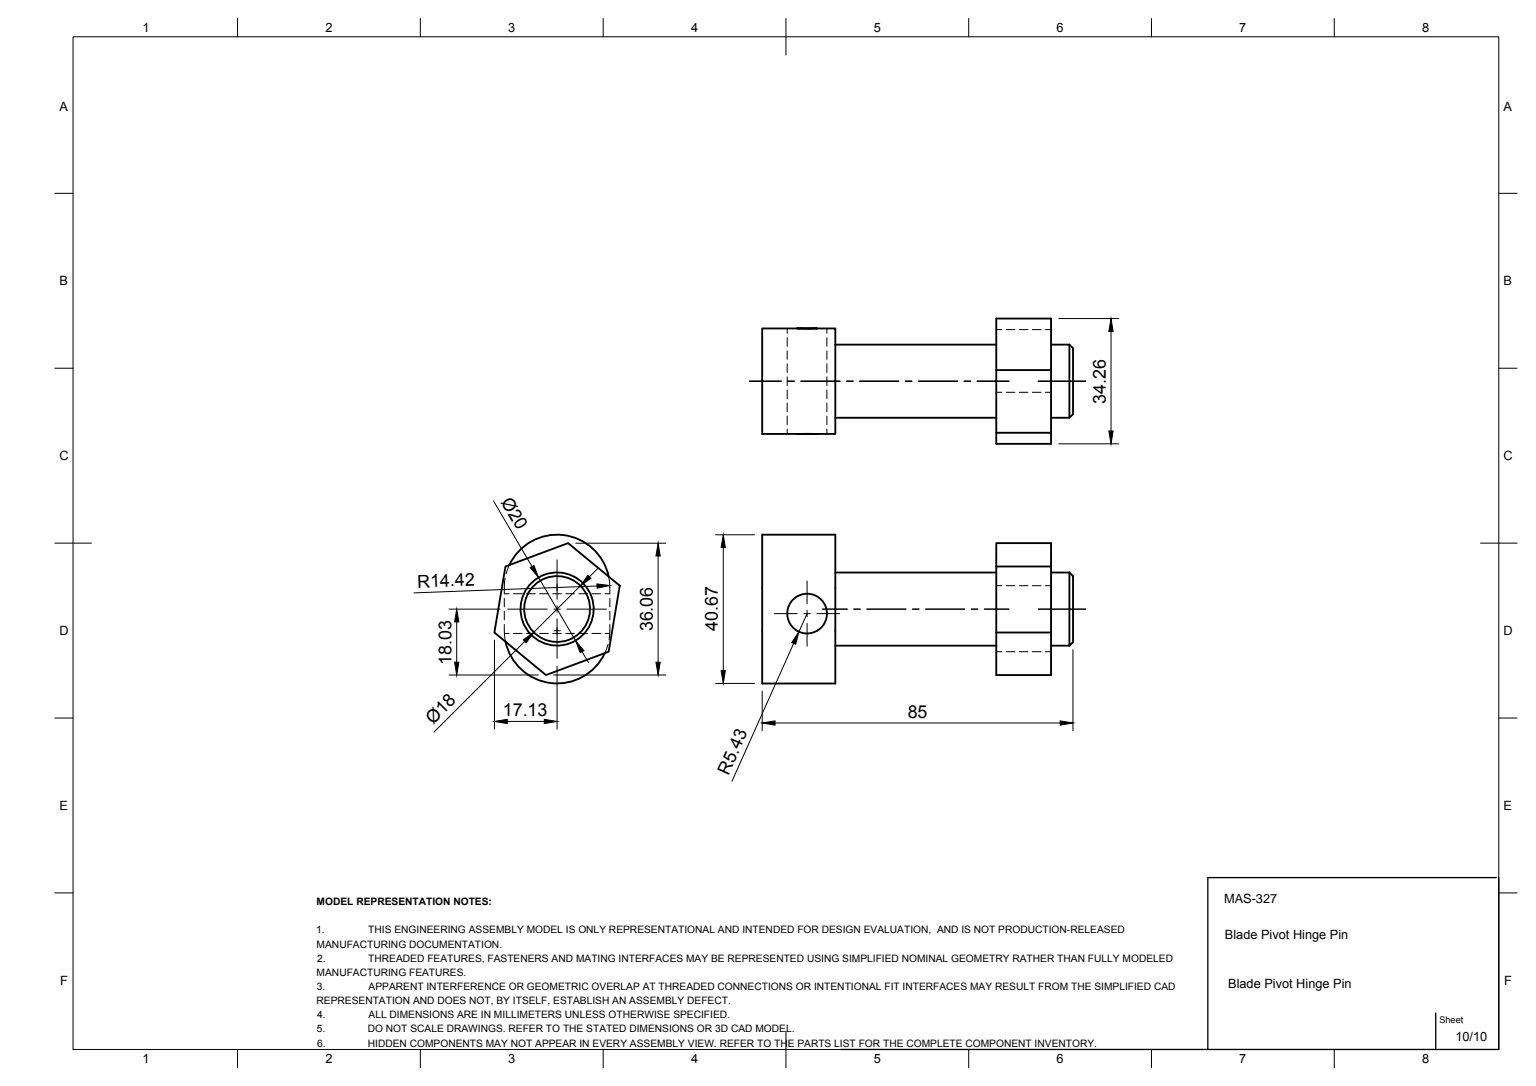
ISO-10303-21;
HEADER;
FILE_DESCRIPTION (('STEP AP214'),
    '1' );
FILE_NAME ('Blade Pivot Hinge Pin.step',
    '2026-10-06T22:16:42',
    ( '' ),
    ( '' ),
    'SwSTEP 2.0',
    'SolidWorks 2025',
    '' );
FILE_SCHEMA (( 'AUTOMOTIVE_DESIGN' ));
ENDSEC;

DATA;
#32=VERTEX_POINT ( 'NONE', #9176 ) ;
#71=CIRCLE ( 'NONE', #14485, 14.42424326798555434 ) ;
#91=AXIS2_PLACEMENT_3D ( 'NONE', #5623, #16792, #1591 ) ;
#93=ORIENTED_EDGE ( 'NONE', *, *, #5608, .T. ) ;
#149=ORIENTED_EDGE ( 'NONE', *, *, #5345, .F. ) ;
#155=FILL_AREA_STYLE_COLOUR ( '', #636 ) ;
#175=VERTEX_POINT ( 'NONE', #1443 ) ;
#180=CARTESIAN_POINT ( 'NONE',  ( 165.8083469658213005, 192.9029763258799335, -44.99999999999997158 ) ) ;
#237=DIRECTION ( 'NONE',  ( 0.000000000000000000, 0.000000000000000000, 1.000000000000000000 ) ) ;
#291=CARTESIAN_POINT ( 'NONE',  ( 163.1026836591718734, 192.4288937294299160, 34.00000000000001421 ) ) ;
#292=CARTESIAN_POINT ( 'NONE',  ( 163.3401611601854029, 191.7221236944928364, 21.73429951086134082 ) ) ;
#367=ORIENTED_EDGE ( 'NONE', *, *, #11936, .F. ) ;
#369=EDGE_LOOP ( 'NONE', ( #21532, #16154, #367, #8720 ) ) ;
#378=LINE ( 'NONE', #18569, #11533 ) ;
#385=CARTESIAN_POINT ( 'NONE',  ( 147.5268905834513475, 193.0332408774651185, -50.99999999999998579 ) ) ;
#410=CARTESIAN_POINT ( 'NONE',  ( 145.5008360144876747, 198.5836349573982886, 14.00000000000001776 ) ) ;
#412=LINE ( 'NONE', #12191, #11898 ) ;
#430=CYLINDRICAL_SURFACE ( 'NONE', #1907, 10.00000000000000888 ) ;
#439=LINE ( 'NONE', #539, #1132 ) ;
#444=DIRECTION ( 'NONE',  ( -0.000000000000000000, -0.000000000000000000, 1.000000000000000000 ) ) ;
#445=ORIENTED_EDGE ( 'NONE', *, *, #15692, .F. ) ;
#457=LINE ( 'NONE', #7188, #7476 ) ;
#497=VERTEX_POINT ( 'NONE', #9152 ) ;
#520=FACE_OUTER_BOUND ( 'NONE', #589, .T. ) ;
#539=CARTESIAN_POINT ( 'NONE',  ( 138.4989748031516967, 208.9305787985672680, -44.99999999999997158 ) ) ;
#583=VECTOR ( 'NONE', #3604, 1000.000000000000114 ) ;
#589=EDGE_LOOP ( 'NONE', ( #10743, #2541, #5246, #20217, #1667 ) ) ;
#612=VECTOR ( 'NONE', #11258, 1000.000000000000227 ) ;
#636=COLOUR_RGB ( '', 0.72549020, 0.75294118, 0.79215686) ;
#692=DIRECTION ( 'NONE',  ( -1.000000000000000000, 0.000000000000000000, 0.000000000000000000 ) ) ;
#696=DIRECTION ( 'NONE',  ( 0.9999746145782334450, -0.007125320983191549967, 0.000000000000000000 ) ) ;
#707=FACE_OUTER_BOUND ( 'NONE', #3120, .T. ) ;
#743=CARTESIAN_POINT ( 'NONE',  ( 157.5268905834513475, 193.0332408774651185, -50.99999999999998579 ) ) ;
#765=CARTESIAN_POINT ( 'NONE',  ( 136.0032066456581390, 182.5367998656340944, 34.00000000000001421 ) ) ;
#804=CYLINDRICAL_SURFACE ( 'NONE', #5889, 10.00000000000000888 ) ;
#883=FACE_OUTER_BOUND ( 'NONE', #16754, .T. ) ;
#884=LINE ( 'NONE', #9271, #9392 ) ;
#886=DIRECTION ( 'NONE',  ( -1.000000000000000000, 0.000000000000000000, 0.000000000000000000 ) ) ;
#956=CIRCLE ( 'NONE', #2372, 5.425037101889737201 ) ;
#973=CARTESIAN_POINT ( 'NONE',  ( 156.5548063637509415, 177.1359029563629406, -29.99999999999997868 ) ) ;
#980=EDGE_CURVE ( 'NONE', #32, #12851, #19907, .T. ) ;
#1057=CARTESIAN_POINT ( 'NONE',  ( 147.5268905834513475, 193.0332408774651185, -50.99999999999998579 ) ) ;
#1061=ADVANCED_FACE ( 'NONE', ( #2071, #9126 ), #20695, .F. ) ;
#1115=ADVANCED_FACE ( 'NONE', ( #520 ), #15825, .T. ) ;
#1122=LINE ( 'NONE', #12914, #6565 ) ;
#1123=VECTOR ( 'NONE', #20357, 1000.000000000000000 ) ;
#1132=VECTOR ( 'NONE', #18955, 1000.000000000000114 ) ;
#1210=FACE_OUTER_BOUND ( 'NONE', #15224, .T. ) ;
#1211=VECTOR ( 'NONE', #3473, 1000.000000000000000 ) ;
#1227=VERTEX_POINT ( 'NONE', #4367 ) ;
#1256=EDGE_CURVE ( 'NONE', #2768, #6341, #16602, .T. ) ;
#1325=ORIENTED_EDGE ( 'NONE', *, *, #18533, .F. ) ;
#1386=EDGE_CURVE ( 'NONE', #6341, #2204, #8241, .T. ) ;
#1395=CYLINDRICAL_SURFACE ( 'NONE', #20750, 14.42424326798555434 ) ;
#1410=PRODUCT_DEFINITION_FORMATION_WITH_SPECIFIED_SOURCE ( 'ANY', '', #14993, .NOT_KNOWN. ) ;
#1418=ORIENTED_EDGE ( 'NONE', *, *, #7944, .F. ) ;
#1420=CARTESIAN_POINT ( 'NONE',  ( 137.5268905834513191, 193.0332408774651185, -29.99999999999997868 ) ) ;
#1429=DIRECTION ( 'NONE',  ( 0.000000000000000000, 0.000000000000000000, -1.000000000000000000 ) ) ;
#1443=CARTESIAN_POINT ( 'NONE',  ( 129.2454342010813662, 193.1635054290503319, -44.99999999999997158 ) ) ;
#1462=EDGE_CURVE ( 'NONE', #9423, #12336, #15502, .T. ) ;
#1473=ORIENTED_EDGE ( 'NONE', *, *, #15351, .T. ) ;
#1537=CARTESIAN_POINT ( 'NONE',  ( 165.8083469658213005, 192.9029763258799335, -44.99999999999997158 ) ) ;
#1561=EDGE_CURVE ( 'NONE', #6540, #20418, #2056, .T. ) ;
#1591=DIRECTION ( 'NONE',  ( -1.000000000000000000, 0.000000000000000000, -0.000000000000000000 ) ) ;
#1613=AXIS2_PLACEMENT_3D ( 'NONE', #14650, #9274, #21390 ) ;
#1667=ORIENTED_EDGE ( 'NONE', *, *, #1675, .T. ) ;
#1675=EDGE_CURVE ( 'NONE', #16415, #5871, #2693, .T. ) ;
#1676=VECTOR ( 'NONE', #18323, 1000.000000000000000 ) ;
#1697=EDGE_CURVE ( 'NONE', #15900, #2204, #8782, .T. ) ;
#1699=VERTEX_POINT ( 'NONE', #2375 ) ;
#1720=SHAPE_REPRESENTATION ( 'Blade Pivot Hinge Pin', ( #12657 ), #4220 ) ;
#1739=ADVANCED_FACE ( 'NONE', ( #20787 ), #16724, .T. ) ;
#1774=ORIENTED_EDGE ( 'NONE', *, *, #5185, .T. ) ;
#1812=CARTESIAN_POINT ( 'NONE',  ( 156.5548063637509415, 177.1359029563629406, -44.99999999999997158 ) ) ;
#1813=CARTESIAN_POINT ( 'NONE',  ( 147.5268905834513475, 193.0332408774651185, -49.99999999999997158 ) ) ;
#1843=( NAMED_UNIT ( * ) PLANE_ANGLE_UNIT ( ) SI_UNIT ( $, .RADIAN. ) );
#1857=EDGE_CURVE ( 'NONE', #16415, #13585, #20018, .T. ) ;
#1864=CARTESIAN_POINT ( 'NONE',  ( 163.1026836591718734, 192.4288937294299160, 34.00000000000001421 ) ) ;
#1907=AXIS2_PLACEMENT_3D ( 'NONE', #20385, #15625, #15526 ) ;
#1933=VERTEX_POINT ( 'NONE', #7782 ) ;
#1948=VECTOR ( 'NONE', #7134, 1000.000000000000227 ) ;
#1991=AXIS2_PLACEMENT_3D ( 'NONE', #5809, #10997, #17814 ) ;
#1993=CIRCLE ( 'NONE', #19956, 14.42424326798555434 ) ;
#2004=LINE ( 'NONE', #20415, #5529 ) ;
#2031=DIRECTION ( 'NONE',  ( 0.3428981916074316239, -0.9393725726208708160, -0.000000000000000000 ) ) ;
#2056=LINE ( 'NONE', #11750, #15327 ) ;
#2071=FACE_OUTER_BOUND ( 'NONE', #10103, .T. ) ;
#2081=CARTESIAN_POINT ( 'NONE',  ( 156.5548063637509415, 177.1359029563629406, -44.99999999999997158 ) ) ;
#2096=DIRECTION ( 'NONE',  ( -0.3428981916074316239, 0.9393725726208708160, 0.000000000000000000 ) ) ;
#2105=ADVANCED_FACE ( 'NONE', ( #21775 ), #12052, .F. ) ;
#2124=ORIENTED_EDGE ( 'NONE', *, *, #21477, .F. ) ;
#2204=VERTEX_POINT ( 'NONE', #13707 ) ;
#2211=EDGE_CURVE ( 'NONE', #13585, #16648, #10200, .T. ) ;
#2284=ADVANCED_FACE ( 'NONE', ( #1210 ), #7217, .T. ) ;
#2303=PLANE ( 'NONE',  #16261 ) ;
#2304=EDGE_CURVE ( 'NONE', #15900, #1933, #11111, .T. ) ;
#2319=DIRECTION ( 'NONE',  ( -1.000000000000000000, 0.000000000000000000, 0.000000000000000000 ) ) ;
#2346=DIRECTION ( 'NONE',  ( -0.007125320983191549967, -0.9999746145782334450, 0.000000000000000000 ) ) ;
#2372=AXIS2_PLACEMENT_3D ( 'NONE', #17761, #9738, #18092 ) ;
#2375=CARTESIAN_POINT ( 'NONE',  ( 136.0032066456581674, 182.5367998656340944, 18.98992973508700643 ) ) ;
#2394=AXIS2_PLACEMENT_3D ( 'NONE', #3060, #9903, #4940 ) ;
#2403=CARTESIAN_POINT ( 'NONE',  ( 0.000000000000000000, 0.000000000000000000, 0.000000000000000000 ) ) ;
#2443=ORIENTED_EDGE ( 'NONE', *, *, #20870, .T. ) ;
#2461=ORIENTED_EDGE ( 'NONE', *, *, #21477, .T. ) ;
#2463=CARTESIAN_POINT ( 'NONE',  ( 138.2733499813809885, 177.2661675079481540, -29.99999999999997868 ) ) ;
#2488=ORIENTED_EDGE ( 'NONE', *, *, #1675, .F. ) ;
#2499=LINE ( 'NONE', #743, #5251 ) ;
#2541=ORIENTED_EDGE ( 'NONE', *, *, #10210, .T. ) ;
#2569=ORIENTED_EDGE ( 'NONE', *, *, #16333, .F. ) ;
#2573=LINE ( 'NONE', #5773, #19594 ) ;
#2583=CARTESIAN_POINT ( 'NONE',  ( 136.1559806577886036, 182.1353248703794350, 23.62031749096655275 ) ) ;
#2667=ORIENTED_EDGE ( 'NONE', *, *, #5537, .T. ) ;
#2674=CARTESIAN_POINT ( 'NONE',  ( 147.5268905834513475, 193.0332408774651185, -44.99999999999997158 ) ) ;
#2693=LINE ( 'NONE', #7565, #6529 ) ;
#2715=AXIS2_PLACEMENT_3D ( 'NONE', #9298, #2346, #696 ) ;
#2768=VERTEX_POINT ( 'NONE', #5833 ) ;
#2806=DIRECTION ( 'NONE',  ( -0.000000000000000000, -0.000000000000000000, -1.000000000000000000 ) ) ;
#2887=PLANE ( 'NONE',  #7204 ) ;
#2914=DIRECTION ( 'NONE',  ( 0.9393725726208708160, 0.3428981916074316794, -0.000000000000000000 ) ) ;
#3026=DIRECTION ( 'NONE',  ( -0.4938165983075539223, 0.8695660798558991766, 0.000000000000000000 ) ) ;
#3060=CARTESIAN_POINT ( 'NONE',  ( 147.5268905834513475, 193.0332408774651185, 14.00000000000001776 ) ) ;
#3120=EDGE_LOOP ( 'NONE', ( #3971, #3699, #6691, #12257 ) ) ;
#3133=CARTESIAN_POINT ( 'NONE',  ( 156.5548063637509415, 177.1359029563629406, -29.99999999999997868 ) ) ;
#3229=EDGE_CURVE ( 'NONE', #12336, #6852, #3737, .T. ) ;
#3237=ORIENTED_EDGE ( 'NONE', *, *, #5860, .T. ) ;
#3248=SURFACE_STYLE_USAGE ( .BOTH. , #6887 ) ;
#3260=EDGE_LOOP ( 'NONE', ( #6641, #16425, #15413, #4890, #20873, #14634, #7629 ) ) ;
#3285=EDGE_CURVE ( 'NONE', #9423, #15135, #21427, .T. ) ;
#3330=EDGE_CURVE ( 'NONE', #12794, #19825, #7275, .T. ) ;
#3384=CARTESIAN_POINT ( 'NONE',  ( 163.1026836591718734, 192.4288937294299160, 34.00000000000001421 ) ) ;
#3404=AXIS2_PLACEMENT_3D ( 'NONE', #14232, #14124, #7424 ) ;
#3406=ORIENTED_EDGE ( 'NONE', *, *, #16132, .F. ) ;
#3407=CARTESIAN_POINT ( 'NONE',  ( 137.5268905834513191, 193.0332408774651185, 14.00000000000001776 ) ) ;
#3420=DIRECTION ( 'NONE',  ( -0.9393725726208708160, -0.3428981916074316239, 0.000000000000000000 ) ) ;
#3464=CIRCLE ( 'NONE', #2394, 10.00000000000000888 ) ;
#3467=EDGE_CURVE ( 'NONE', #5871, #8301, #1993, .T. ) ;
#3473=DIRECTION ( 'NONE',  ( 0.7071067811865456854, 0.000000000000000000, 0.7071067811865493491 ) ) ;
#3497=CARTESIAN_POINT ( 'NONE',  ( 129.2454342010813662, 193.1635054290503319, -29.99999999999997868 ) ) ;
#3540=ORIENTED_EDGE ( 'NONE', *, *, #18228, .F. ) ;
#3553=PRODUCT_DEFINITION_CONTEXT ( 'detailed design', #11668, 'design' ) ;
#3576=FACE_BOUND ( 'NONE', #8312, .T. ) ;
#3587=LINE ( 'NONE', #17017, #10630 ) ;
#3604=DIRECTION ( 'NONE',  ( -0.3428981916074316239, 0.9393725726208708160, 0.000000000000000000 ) ) ;
#3633=PLANE ( 'NONE',  #19511 ) ;
#3646=EDGE_CURVE ( 'NONE', #12851, #32, #3464, .T. ) ;
#3661=CARTESIAN_POINT ( 'NONE',  ( 138.5268905834513191, 193.0332408774651185, -50.99999999999998579 ) ) ;
#3699=ORIENTED_EDGE ( 'NONE', *, *, #14722, .F. ) ;
#3701=ORIENTED_EDGE ( 'NONE', *, *, #15830, .F. ) ;
#3737=LINE ( 'NONE', #2081, #14645 ) ;
#3785=AXIS2_PLACEMENT_3D ( 'NONE', #1057, #19682, #21452 ) ;
#3810=AXIS2_PLACEMENT_3D ( 'NONE', #10387, #6975, #17304 ) ;
#3856=AXIS2_PLACEMENT_3D ( 'NONE', #9588, #21159, #4387 ) ;
#3861=ORIENTED_EDGE ( 'NONE', *, *, #15351, .F. ) ;
#3895=FACE_OUTER_BOUND ( 'NONE', #4743, .T. ) ;
#3906=ORIENTED_EDGE ( 'NONE', *, *, #980, .F. ) ;
#3921=CARTESIAN_POINT ( 'NONE',  ( 163.3215298332769407, 191.7840731147956319, 22.69574685642843193 ) ) ;
#3935=EDGE_CURVE ( 'NONE', #14777, #14246, #412, .T. ) ;
#3971=ORIENTED_EDGE ( 'NONE', *, *, #5276, .T. ) ;
#4000=CARTESIAN_POINT ( 'NONE',  ( 131.9510975077307933, 193.6375880255003779, 14.00000000000001776 ) ) ;
#4008=LINE ( 'NONE', #4219, #19072 ) ;
#4049=EDGE_LOOP ( 'NONE', ( #10376, #18796, #8509, #20618 ) ) ;
#4074=ORIENTED_EDGE ( 'NONE', *, *, #5608, .F. ) ;
#4094=ORIENTED_EDGE ( 'NONE', *, *, #8231, .T. ) ;
#4136=CIRCLE ( 'NONE', #4292, 10.00000000000000888 ) ;
#4158=ORIENTED_EDGE ( 'NONE', *, *, #17674, .F. ) ;
#4219=CARTESIAN_POINT ( 'NONE',  ( 136.0032066456581390, 182.5367998656340944, 34.00000000000001421 ) ) ;
#4220=( GEOMETRIC_REPRESENTATION_CONTEXT ( 3 ) GLOBAL_UNCERTAINTY_ASSIGNED_CONTEXT ( ( #20336 ) ) GLOBAL_UNIT_ASSIGNED_CONTEXT ( ( #21579, #1843, #6470 ) ) REPRESENTATION_CONTEXT ( 'NONE', 'WORKASPACE' ) );
#4251=ORIENTED_EDGE ( 'NONE', *, *, #3330, .F. ) ;
#4255=DIRECTION ( 'NONE',  ( -1.000000000000000000, 0.000000000000000000, -0.000000000000000000 ) ) ;
#4261=DIRECTION ( 'NONE',  ( -1.000000000000000000, 0.000000000000000000, 0.000000000000000000 ) ) ;
#4292=AXIS2_PLACEMENT_3D ( 'NONE', #10711, #17414, #2319 ) ;
#4304=ORIENTED_EDGE ( 'NONE', *, *, #7932, .F. ) ;
#4323=VERTEX_POINT ( 'NONE', #4574 ) ;
#4329=DIRECTION ( 'NONE',  ( -1.000000000000000000, 0.000000000000000000, 0.000000000000000000 ) ) ;
#4330=CARTESIAN_POINT ( 'NONE',  ( 165.8083469658213005, 192.9029763258799335, -29.99999999999997868 ) ) ;
#4367=CARTESIAN_POINT ( 'NONE',  ( 138.4989748031516967, 208.9305787985672680, -29.99999999999997868 ) ) ;
#4387=DIRECTION ( 'NONE',  ( -1.000000000000000000, 0.000000000000000000, 0.000000000000000000 ) ) ;
#4463=EDGE_CURVE ( 'NONE', #10265, #14309, #19983, .T. ) ;
#4530=DIRECTION ( 'NONE',  ( 0.4938165983075534227, -0.8695660798558993987, 0.000000000000000000 ) ) ;
#4574=CARTESIAN_POINT ( 'NONE',  ( 159.6377923430271153, 201.9209935688625421, 21.73429951086134082 ) ) ;
#4582=LINE ( 'NONE', #6463, #12990 ) ;
#4597=CARTESIAN_POINT ( 'NONE',  ( 145.5008360144876747, 198.5836349573982886, 34.00000000000001421 ) ) ;
#4627=ORIENTED_EDGE ( 'NONE', *, *, #11087, .T. ) ;
#4658=EDGE_LOOP ( 'NONE', ( #12688, #8306, #8008, #21182 ) ) ;
#4673=CARTESIAN_POINT ( 'NONE',  ( 138.2733499813809885, 177.2661675079481540, -44.99999999999997158 ) ) ;
#4699=CARTESIAN_POINT ( 'NONE',  ( 163.3023584364855196, 191.8436256089667324, 20.54250398750395590 ) ) ;
#4721=DIRECTION ( 'NONE',  ( -0.000000000000000000, -0.000000000000000000, 1.000000000000000000 ) ) ;
#4743=EDGE_LOOP ( 'NONE', ( #19322, #8584, #17876, #20034 ) ) ;
#4817=AXIS2_PLACEMENT_3D ( 'NONE', #11281, #2914, #6327 ) ;
#4829=EDGE_LOOP ( 'NONE', ( #2443, #18990, #4158, #18962 ) ) ;
#4835=CARTESIAN_POINT ( 'NONE',  ( 163.3401611601854029, 191.7221236944928364, 21.73429951086134082 ) ) ;
#4837=ADVANCED_FACE ( 'NONE', ( #707 ), #7440, .F. ) ;
#4860=VERTEX_POINT ( 'NONE', #20125 ) ;
#4890=ORIENTED_EDGE ( 'NONE', *, *, #16132, .T. ) ;
#4930=CARTESIAN_POINT ( 'NONE',  ( 177.7722984847500527, 196.9902717476302882, 21.73429951086134082 ) ) ;
#4940=DIRECTION ( 'NONE',  ( -1.000000000000000000, 0.000000000000000000, 0.000000000000000000 ) ) ;
#4979=PRODUCT_DEFINITION_SHAPE ( 'NONE', 'NONE',  #8803 ) ;
#4988=DIRECTION ( 'NONE',  ( -0.000000000000000000, -0.000000000000000000, 1.000000000000000000 ) ) ;
#5012=VECTOR ( 'NONE', #444, 1000.000000000000000 ) ;
#5015=CARTESIAN_POINT ( 'NONE',  ( 163.1026836591718734, 192.4288937294299160, 24.47866928663567521 ) ) ;
#5020=CARTESIAN_POINT ( 'NONE',  ( 165.8083469658213005, 192.9029763258799335, -29.99999999999997868 ) ) ;
#5033=ADVANCED_FACE ( 'NONE', ( #10629 ), #804, .T. ) ;
#5052=CARTESIAN_POINT ( 'NONE',  ( 147.5268905834513475, 193.0332408774651185, 14.00000000000001776 ) ) ;
#5095=LINE ( 'NONE', #8408, #6858 ) ;
#5099=ADVANCED_FACE ( 'NONE', ( #20980 ), #15578, .F. ) ;
#5118=( LENGTH_UNIT ( ) NAMED_UNIT ( * ) SI_UNIT ( .MILLI., .METRE. ) );
#5151=DIRECTION ( 'NONE',  ( 0.000000000000000000, 0.000000000000000000, 1.000000000000000000 ) ) ;
#5185=EDGE_CURVE ( 'NONE', #1933, #1699, #956, .T. ) ;
#5221=EDGE_LOOP ( 'NONE', ( #5749, #9154, #20697, #12554 ) ) ;
#5242=CARTESIAN_POINT ( 'NONE',  ( 131.9510975077307933, 193.6375880255003779, 34.00000000000001421 ) ) ;
#5246=ORIENTED_EDGE ( 'NONE', *, *, #5344, .T. ) ;
#5251=VECTOR ( 'NONE', #20916, 1000.000000000000000 ) ;
#5276=EDGE_CURVE ( 'NONE', #10216, #1227, #21197, .T. ) ;
#5324=ORIENTED_EDGE ( 'NONE', *, *, #1386, .T. ) ;
#5344=EDGE_CURVE ( 'NONE', #5609, #497, #9420, .T. ) ;
#5345=EDGE_CURVE ( 'NONE', #1699, #16648, #2004, .T. ) ;
#5374=EDGE_LOOP ( 'NONE', ( #20914, #1325, #7393, #12040 ) ) ;
#5417=AXIS2_PLACEMENT_3D ( 'NONE', #4597, #10012, #13315 ) ;
#5437=EDGE_CURVE ( 'NONE', #175, #10216, #6533, .T. ) ;
#5468=VERTEX_POINT ( 'NONE', #13363 ) ;
#5475=VECTOR ( 'NONE', #2031, 1000.000000000000114 ) ;
#5529=VECTOR ( 'NONE', #18760, 1000.000000000000000 ) ;
#5537=EDGE_CURVE ( 'NONE', #11247, #32, #19298, .T. ) ;
#5563=CARTESIAN_POINT ( 'NONE',  ( 163.3401611601853745, 191.7221236944928364, 22.21121901686272793 ) ) ;
#5608=EDGE_CURVE ( 'NONE', #19825, #12794, #4136, .T. ) ;
#5609=VERTEX_POINT ( 'NONE', #14108 ) ;
#5610=CARTESIAN_POINT ( 'NONE',  ( 138.4989748031516967, 208.9305787985672680, -44.99999999999997158 ) ) ;
#5623=CARTESIAN_POINT ( 'NONE',  ( 0.000000000000000000, 0.000000000000000000, -44.99999999999997158 ) ) ;
#5631=ADVANCED_FACE ( 'NONE', ( #8948 ), #15655, .F. ) ;
#5651=CARTESIAN_POINT ( 'NONE',  ( 136.0451547902032701, 182.4218825594992950, 19.19853326693791473 ) ) ;
#5669=EDGE_CURVE ( 'NONE', #8397, #19825, #457, .T. ) ;
#5740=EDGE_LOOP ( 'NONE', ( #11373, #10373 ) ) ;
#5749=ORIENTED_EDGE ( 'NONE', *, *, #15830, .T. ) ;
#5755=CARTESIAN_POINT ( 'NONE',  ( 136.1510593568410172, 182.1483534088744420, 19.85643285628697541 ) ) ;
#5773=CARTESIAN_POINT ( 'NONE',  ( 174.0518276614676267, 207.1825338655619646, 21.73429951086134082 ) ) ;
#5792=ORIENTED_EDGE ( 'NONE', *, *, #1857, .F. ) ;
#5809=CARTESIAN_POINT ( 'NONE',  ( 156.7804311855217065, 208.8003142469820830, -44.99999999999997158 ) ) ;
#5833=CARTESIAN_POINT ( 'NONE',  ( 163.1026836591718734, 192.4288937294299160, 18.98992973508700643 ) ) ;
#5844=ORIENTED_EDGE ( 'NONE', *, *, #1697, .T. ) ;
#5860=EDGE_CURVE ( 'NONE', #4860, #13585, #71, .T. ) ;
#5871=VERTEX_POINT ( 'NONE', #8794 ) ;
#5889=AXIS2_PLACEMENT_3D ( 'NONE', #15788, #19320, #17334 ) ;
#5943=DIRECTION ( 'NONE',  ( -1.000000000000000000, 0.000000000000000000, 0.000000000000000000 ) ) ;
#6000=PRODUCT_CONTEXT ( 'NONE', #15354, 'mechanical' ) ;
#6053=DIRECTION ( 'NONE',  ( 0.000000000000000000, 0.000000000000000000, -1.000000000000000000 ) ) ;
#6056=DIRECTION ( 'NONE',  ( 0.000000000000000000, 0.000000000000000000, 1.000000000000000000 ) ) ;
#6083=CARTESIAN_POINT ( 'NONE',  ( 129.2454342010813662, 193.1635054290503319, -29.99999999999997868 ) ) ;
#6130=AXIS2_PLACEMENT_3D ( 'NONE', #14301, #17819, #17606 ) ;
#6202=VECTOR ( 'NONE', #20458, 1000.000000000000227 ) ;
#6261=ORIENTED_EDGE ( 'NONE', *, *, #1857, .T. ) ;
#6327=DIRECTION ( 'NONE',  ( 0.3428981916074309577, -0.9393725726208709270, 0.000000000000000000 ) ) ;
#6341=VERTEX_POINT ( 'NONE', #292 ) ;
#6368=DIRECTION ( 'NONE',  ( 0.000000000000000000, 0.000000000000000000, 1.000000000000000000 ) ) ;
#6379=LINE ( 'NONE', #13108, #20764 ) ;
#6417=CYLINDRICAL_SURFACE ( 'NONE', #6993, 10.00000000000000888 ) ;
#6437=EDGE_CURVE ( 'NONE', #8301, #18099, #15396, .T. ) ;
#6463=CARTESIAN_POINT ( 'NONE',  ( 138.4989748031516967, 208.9305787985672680, -29.99999999999997868 ) ) ;
#6470=( NAMED_UNIT ( * ) SI_UNIT ( $, .STERADIAN. ) SOLID_ANGLE_UNIT ( ) );
#6484=AXIS2_PLACEMENT_3D ( 'NONE', #21065, #6056, #12893 ) ;
#6499=FACE_OUTER_BOUND ( 'NONE', #5374, .T. ) ;
#6529=VECTOR ( 'NONE', #12728, 1000.000000000000114 ) ;
#6533=LINE ( 'NONE', #13253, #1676 ) ;
#6540=VERTEX_POINT ( 'NONE', #12509 ) ;
#6554=SURFACE_STYLE_FILL_AREA ( #18456 ) ;
#6565=VECTOR ( 'NONE', #4530, 1000.000000000000114 ) ;
#6608=CARTESIAN_POINT ( 'NONE',  ( 159.0505745212445561, 203.5296818892961994, 14.00000000000001776 ) ) ;
#6641=ORIENTED_EDGE ( 'NONE', *, *, #6437, .T. ) ;
#6657=CARTESIAN_POINT ( 'NONE',  ( 156.7804311855217065, 208.8003142469820830, -29.99999999999997868 ) ) ;
#6671=ORIENTED_EDGE ( 'NONE', *, *, #9508, .T. ) ;
#6681=CARTESIAN_POINT ( 'NONE',  ( 136.0032066456581390, 182.5367998656340944, 14.00000000000001776 ) ) ;
#6690=CARTESIAN_POINT ( 'NONE',  ( 161.4980277546683283, 196.8248625098966897, 21.73429951086134082 ) ) ;
#6691=ORIENTED_EDGE ( 'NONE', *, *, #14114, .F. ) ;
#6707=CARTESIAN_POINT ( 'NONE',  ( 163.3167426812955227, 191.7976672453297624, 20.78115173001200944 ) ) ;
#6723=ORIENTED_EDGE ( 'NONE', *, *, #5537, .F. ) ;
#6752=ORIENTED_EDGE ( 'NONE', *, *, #5669, .T. ) ;
#6763=CARTESIAN_POINT ( 'NONE',  ( 145.5008360144876747, 198.5836349573982886, 34.00000000000001421 ) ) ;
#6787=DIRECTION ( 'NONE',  ( -0.9999746145782334450, 0.007125320983193088667, 0.000000000000000000 ) ) ;
#6789=EDGE_CURVE ( 'NONE', #20418, #4860, #12398, .T. ) ;
#6851=ORIENTED_EDGE ( 'NONE', *, *, #20870, .F. ) ;
#6852=VERTEX_POINT ( 'NONE', #4673 ) ;
#6858=VECTOR ( 'NONE', #18432, 1000.000000000000000 ) ;
#6871=ADVANCED_FACE ( 'NONE', ( #16456, #3576 ), #15032, .T. ) ;
#6887=SURFACE_SIDE_STYLE ('',( #6554 ) ) ;
#6901=AXIS2_PLACEMENT_3D ( 'NONE', #5052, #8480, #15188 ) ;
#6963=ADVANCED_FACE ( 'NONE', ( #16899 ), #8648, .F. ) ;
#6975=DIRECTION ( 'NONE',  ( -0.000000000000000000, -0.000000000000000000, -1.000000000000000000 ) ) ;
#6993=AXIS2_PLACEMENT_3D ( 'NONE', #21639, #4988, #19869 ) ;
#7002=DIRECTION ( 'NONE',  ( 0.3428981916074309577, -0.9393725726208709270, 0.000000000000000000 ) ) ;
#7050=DIRECTION ( 'NONE',  ( 0.000000000000000000, 0.000000000000000000, 1.000000000000000000 ) ) ;
#7102=MANIFOLD_SOLID_BREP ( 'Chamfer1', #13383 ) ;
#7125=VECTOR ( 'NONE', #11815, 1000.000000000000000 ) ;
#7126=CIRCLE ( 'NONE', #15222, 10.00000000000000888 ) ;
#7134=DIRECTION ( 'NONE',  ( -0.5061580162706792452, -0.8624407588727069918, 0.000000000000000000 ) ) ;
#7188=CARTESIAN_POINT ( 'NONE',  ( 137.5268905834513191, 193.0332408774651185, -50.99999999999998579 ) ) ;
#7204=AXIS2_PLACEMENT_3D ( 'NONE', #15996, #11152, #16432 ) ;
#7217=CYLINDRICAL_SURFACE ( 'NONE', #20627, 14.42424326798555434 ) ;
#7224=DIRECTION ( 'NONE',  ( -0.000000000000000000, -0.000000000000000000, -1.000000000000000000 ) ) ;
#7228=ADVANCED_FACE ( 'NONE', ( #6499 ), #12566, .F. ) ;
#7242=CARTESIAN_POINT ( 'NONE',  ( 136.2768881589198600, 181.8432453435729883, 21.97307119874763259 ) ) ;
#7275=CIRCLE ( 'NONE', #19574, 10.00000000000000888 ) ;
#7329=DIRECTION ( 'NONE',  ( -0.000000000000000000, -0.000000000000000000, -1.000000000000000000 ) ) ;
#7348=EDGE_CURVE ( 'NONE', #14309, #10265, #16864, .T. ) ;
#7393=ORIENTED_EDGE ( 'NONE', *, *, #1462, .F. ) ;
#7424=DIRECTION ( 'NONE',  ( 1.000000000000000000, 0.000000000000000000, 0.000000000000000000 ) ) ;
#7433=ORIENTED_EDGE ( 'NONE', *, *, #7932, .T. ) ;
#7440=PLANE ( 'NONE',  #12589 ) ;
#7452=CARTESIAN_POINT ( 'NONE',  ( 163.2639715594360155, 191.9628544139417841, 23.38668371770654275 ) ) ;
#7476=VECTOR ( 'NONE', #17735, 1000.000000000000000 ) ;
#7500=ADVANCED_FACE ( 'NONE', ( #8705 ), #3633, .F. ) ;
#7539=UNCERTAINTY_MEASURE_WITH_UNIT (LENGTH_MEASURE( 1.000000000000000082E-05 ), #5118, 'distance_accuracy_value', 'NONE');
#7543=EDGE_LOOP ( 'NONE', ( #4627, #9285 ) ) ;
#7554=CARTESIAN_POINT ( 'NONE',  ( 156.7804311855217065, 208.8003142469820830, -29.99999999999997868 ) ) ;
#7565=CARTESIAN_POINT ( 'NONE',  ( 136.0032066456581390, 182.5367998656340944, 34.00000000000001421 ) ) ;
#7585=AXIS2_PLACEMENT_3D ( 'NONE', #12636, #19357, #4255 ) ;
#7623=DIRECTION ( 'NONE',  ( -0.000000000000000000, -0.000000000000000000, -1.000000000000000000 ) ) ;
#7629=ORIENTED_EDGE ( 'NONE', *, *, #10210, .F. ) ;
#7645=ADVANCED_FACE ( 'NONE', ( #21259 ), #15952, .F. ) ;
#7767=ORIENTED_EDGE ( 'NONE', *, *, #20655, .F. ) ;
#7769=DIRECTION ( 'NONE',  ( -0.000000000000000000, -0.000000000000000000, 1.000000000000000000 ) ) ;
#7770=DIRECTION ( 'NONE',  ( -0.5061580162706792452, -0.8624407588727069918, 0.000000000000000000 ) ) ;
#7782=CARTESIAN_POINT ( 'NONE',  ( 132.5383153295133809, 192.0288997050666921, 21.73429951086134082 ) ) ;
#7906=DIRECTION ( 'NONE',  ( 0.9999746145782334450, -0.007125320983191549967, 0.000000000000000000 ) ) ;
#7932=EDGE_CURVE ( 'NONE', #16648, #6540, #18152, .T. ) ;
#7944=EDGE_CURVE ( 'NONE', #497, #16415, #20983, .T. ) ;
#7947=VECTOR ( 'NONE', #15174, 1000.000000000000341 ) ;
#8008=ORIENTED_EDGE ( 'NONE', *, *, #3229, .F. ) ;
#8068=ORIENTED_EDGE ( 'NONE', *, *, #6789, .F. ) ;
#8231=EDGE_CURVE ( 'NONE', #2768, #4323, #11182, .T. ) ;
#8241=LINE ( 'NONE', #4930, #7947 ) ;
#8249=DIRECTION ( 'NONE',  ( 0.000000000000000000, 0.000000000000000000, 1.000000000000000000 ) ) ;
#8301=VERTEX_POINT ( 'NONE', #9552 ) ;
#8306=ORIENTED_EDGE ( 'NONE', *, *, #12097, .F. ) ;
#8312=EDGE_LOOP ( 'NONE', ( #4251, #4074 ) ) ;
#8333=DIRECTION ( 'NONE',  ( 0.9393725726208708160, 0.3428981916074316794, -0.000000000000000000 ) ) ;
#8367=CARTESIAN_POINT ( 'NONE',  ( 157.5268905834513475, 193.0332408774651185, -44.99999999999997158 ) ) ;
#8397=VERTEX_POINT ( 'NONE', #21674 ) ;
#8400=ORIENTED_EDGE ( 'NONE', *, *, #2211, .T. ) ;
#8408=CARTESIAN_POINT ( 'NONE',  ( 156.5548063637509415, 177.1359029563629406, -44.99999999999997158 ) ) ;
#8440=DIRECTION ( 'NONE',  ( 0.5061580162706794672, 0.8624407588727069918, 0.000000000000000000 ) ) ;
#8442=AXIS2_PLACEMENT_3D ( 'NONE', #1537, #14862, #11666 ) ;
#8480=DIRECTION ( 'NONE',  ( 0.000000000000000000, 0.000000000000000000, -1.000000000000000000 ) ) ;
#8507=ORIENTED_EDGE ( 'NONE', *, *, #2211, .F. ) ;
#8509=ORIENTED_EDGE ( 'NONE', *, *, #20655, .T. ) ;
#8524=LINE ( 'NONE', #6657, #17999 ) ;
#8584=ORIENTED_EDGE ( 'NONE', *, *, #15692, .T. ) ;
#8624=FACE_OUTER_BOUND ( 'NONE', #8885, .T. ) ;
#8648=PLANE ( 'NONE',  #15227 ) ;
#8660=DIRECTION ( 'NONE',  ( 1.000000000000000000, 0.000000000000000000, 0.000000000000000000 ) ) ;
#8670=AXIS2_PLACEMENT_3D ( 'NONE', #9901, #8249, #21697 ) ;
#8705=FACE_OUTER_BOUND ( 'NONE', #3260, .T. ) ;
#8720=ORIENTED_EDGE ( 'NONE', *, *, #12097, .T. ) ;
#8782=B_SPLINE_CURVE_WITH_KNOTS ( 'NONE', 3,
 ( #12513, #19452, #2583, #12402, #17785, #17464, #7242, #19134 ),
 .UNSPECIFIED., .F., .F.,
 ( 4, 2, 2, 4 ),
 ( 3.469446951953614189E-18, 0.001432241572422971983, 0.002148362358634445940, 0.002864483144845920114 ),
 .UNSPECIFIED. ) ;
#8794=CARTESIAN_POINT ( 'NONE',  ( 136.0032066456581390, 182.5367998656340944, 34.00000000000001421 ) ) ;
#8803=PRODUCT_DEFINITION ( 'UNKNOWN', '', #1410, #3553 ) ;
#8812=DIRECTION ( 'NONE',  ( -0.9999746145782334450, 0.007125320983193089534, 0.000000000000000000 ) ) ;
#8885=EDGE_LOOP ( 'NONE', ( #1473, #5844, #18307, #9332, #7433, #3406, #10717, #10721, #19853, #16558 ) ) ;
#8936=ADVANCED_FACE ( 'NONE', ( #18090 ), #6417, .T. ) ;
#8948=FACE_OUTER_BOUND ( 'NONE', #19887, .T. ) ;
#8972=CARTESIAN_POINT ( 'NONE',  ( 136.2768881589198884, 181.8432453435730167, 21.73429951086134082 ) ) ;
#8977=ORIENTED_EDGE ( 'NONE', *, *, #16333, .T. ) ;
#9016=ORIENTED_EDGE ( 'NONE', *, *, #11936, .T. ) ;
#9080=DIRECTION ( 'NONE',  ( 0.000000000000000000, 0.000000000000000000, 1.000000000000000000 ) ) ;
#9102=DIRECTION ( 'NONE',  ( -0.9393725726208707050, -0.3428981916074316239, -0.000000000000000000 ) ) ;
#9126=FACE_BOUND ( 'NONE', #7543, .T. ) ;
#9152=CARTESIAN_POINT ( 'NONE',  ( 131.0765927465021434, 198.5836349573982886, 34.00000000000001421 ) ) ;
#9154=ORIENTED_EDGE ( 'NONE', *, *, #3285, .F. ) ;
#9167=FACE_BOUND ( 'NONE', #15105, .T. ) ;
#9170=DIRECTION ( 'NONE',  ( -0.000000000000000000, -0.000000000000000000, 1.000000000000000000 ) ) ;
#9173=ORIENTED_EDGE ( 'NONE', *, *, #1561, .F. ) ;
#9175=ADVANCED_FACE ( 'NONE', ( #8624 ), #19084, .T. ) ;
#9176=CARTESIAN_POINT ( 'NONE',  ( 157.5268905834513475, 193.0332408774651185, 14.00000000000001776 ) ) ;
#9270=( NAMED_UNIT ( * ) PLANE_ANGLE_UNIT ( ) SI_UNIT ( $, .RADIAN. ) );
#9271=CARTESIAN_POINT ( 'NONE',  ( 159.0505745212445561, 203.5296818892961994, 34.00000000000001421 ) ) ;
#9274=DIRECTION ( 'NONE',  ( -0.9393725726208707050, -0.3428981916074317349, 0.000000000000000000 ) ) ;
#9285=ORIENTED_EDGE ( 'NONE', *, *, #20323, .T. ) ;
#9298=CARTESIAN_POINT ( 'NONE',  ( 138.4989748031516967, 208.9305787985672680, -44.99999999999997158 ) ) ;
#9332=ORIENTED_EDGE ( 'NONE', *, *, #5345, .T. ) ;
#9381=DIRECTION ( 'NONE',  ( -0.000000000000000000, -0.000000000000000000, -1.000000000000000000 ) ) ;
#9392=VECTOR ( 'NONE', #7623, 1000.000000000000000 ) ;
#9407=VECTOR ( 'NONE', #9865, 1000.000000000000114 ) ;
#9420=CIRCLE ( 'NONE', #21741, 14.42424326798555434 ) ;
#9423=VERTEX_POINT ( 'NONE', #12894 ) ;
#9474=DIRECTION ( 'NONE',  ( -1.000000000000000000, 0.000000000000000000, 0.000000000000000000 ) ) ;
#9508=EDGE_CURVE ( 'NONE', #5609, #20418, #884, .T. ) ;
#9552=CARTESIAN_POINT ( 'NONE',  ( 163.1026836591718734, 192.4288937294299160, 34.00000000000001421 ) ) ;
#9568=CARTESIAN_POINT ( 'NONE',  ( 163.1026836591718734, 192.4288937294299160, 18.98992973508700643 ) ) ;
#9588=CARTESIAN_POINT ( 'NONE',  ( 147.5268905834513475, 193.0332408774651185, -29.99999999999997868 ) ) ;
#9738=DIRECTION ( 'NONE',  ( -0.9393725726208707050, -0.3428981916074317349, 0.000000000000000000 ) ) ;
#9759=CARTESIAN_POINT ( 'NONE',  ( 145.5008360144876747, 198.5836349573982886, 14.00000000000001776 ) ) ;
#9865=DIRECTION ( 'NONE',  ( -0.9999746145782334450, 0.007125320983193089534, 0.000000000000000000 ) ) ;
#9877=ORIENTED_EDGE ( 'NONE', *, *, #21484, .F. ) ;
#9894=CARTESIAN_POINT ( 'NONE',  ( 163.1866912085270371, 192.1987543186987466, 19.40769008390923389 ) ) ;
#9901=CARTESIAN_POINT ( 'NONE',  ( 149.5529451524149920, 187.4828467975320336, 14.00000000000001776 ) ) ;
#9903=DIRECTION ( 'NONE',  ( 0.000000000000000000, 0.000000000000000000, -1.000000000000000000 ) ) ;
#9922=DIRECTION ( 'NONE',  ( -1.000000000000000000, 0.000000000000000000, 0.000000000000000000 ) ) ;
#9989=DIRECTION ( 'NONE',  ( 0.3428981916074309577, -0.9393725726208709270, 0.000000000000000000 ) ) ;
#9996=ORIENTED_EDGE ( 'NONE', *, *, #20323, .F. ) ;
#9999=ADVANCED_FACE ( 'NONE', ( #20928 ), #11101, .F. ) ;
#10012=DIRECTION ( 'NONE',  ( 0.000000000000000000, 0.000000000000000000, 1.000000000000000000 ) ) ;
#10059=AXIS2_PLACEMENT_3D ( 'NONE', #10870, #17572, #13944 ) ;
#10103=EDGE_LOOP ( 'NONE', ( #16553, #20528, #18905, #19844, #3701, #6851 ) ) ;
#10142=DIRECTION ( 'NONE',  ( 0.3428981916074316239, -0.9393725726208708160, 0.000000000000000000 ) ) ;
#10200=LINE ( 'NONE', #6681, #5475 ) ;
#10210=EDGE_CURVE ( 'NONE', #8301, #5609, #21795, .T. ) ;
#10216=VERTEX_POINT ( 'NONE', #3497 ) ;
#10265=VERTEX_POINT ( 'NONE', #10652 ) ;
#10281=CARTESIAN_POINT ( 'NONE',  ( 136.0032066456581390, 182.5367998656340944, 24.47866928663567521 ) ) ;
#10308=DIRECTION ( 'NONE',  ( 0.8624407588727069918, -0.5061580162706794672, 0.000000000000000000 ) ) ;
#10339=DIRECTION ( 'NONE',  ( -0.000000000000000000, -0.000000000000000000, 1.000000000000000000 ) ) ;
#10344=ORIENTED_EDGE ( 'NONE', *, *, #5185, .F. ) ;
#10368=CIRCLE ( 'NONE', #16339, 10.00000000000000888 ) ;
#10373=ORIENTED_EDGE ( 'NONE', *, *, #7348, .T. ) ;
#10376=ORIENTED_EDGE ( 'NONE', *, *, #5669, .F. ) ;
#10387=CARTESIAN_POINT ( 'NONE',  ( 149.5529451524149920, 187.4828467975320336, 34.00000000000001421 ) ) ;
#10515=MECHANICAL_DESIGN_GEOMETRIC_PRESENTATION_REPRESENTATION('',(#21413),#20361);
#10518=EDGE_CURVE ( 'NONE', #17794, #16883, #18001, .T. ) ;
#10521=CARTESIAN_POINT ( 'NONE',  ( 136.0032066456581674, 182.5367998656340944, 18.98992973508700643 ) ) ;
#10629=FACE_OUTER_BOUND ( 'NONE', #4049, .T. ) ;
#10630=VECTOR ( 'NONE', #15687, 1000.000000000000000 ) ;
#10643=ORIENTED_EDGE ( 'NONE', *, *, #1697, .F. ) ;
#10652=CARTESIAN_POINT ( 'NONE',  ( 156.5268905834513475, 193.0332408774651185, -50.99999999999998579 ) ) ;
#10711=CARTESIAN_POINT ( 'NONE',  ( 147.5268905834513475, 193.0332408774651185, -44.99999999999997158 ) ) ;
#10717=ORIENTED_EDGE ( 'NONE', *, *, #1256, .T. ) ;
#10721=ORIENTED_EDGE ( 'NONE', *, *, #21484, .T. ) ;
#10743=ORIENTED_EDGE ( 'NONE', *, *, #3467, .T. ) ;
#10755=CARTESIAN_POINT ( 'NONE',  ( 163.1026836591718734, 192.4288937294299160, 24.47866928663567521 ) ) ;
#10773=EDGE_CURVE ( 'NONE', #4323, #18099, #19251, .T. ) ;
#10870=CARTESIAN_POINT ( 'NONE',  ( 147.5268905834513475, 193.0332408774651185, -50.99999999999998579 ) ) ;
#10872=SHAPE_DEFINITION_REPRESENTATION ( #4979, #1720 ) ;
#10997=DIRECTION ( 'NONE',  ( -0.8695660798558993987, -0.4938165983075534782, 0.000000000000000000 ) ) ;
#11087=EDGE_CURVE ( 'NONE', #11247, #20292, #18190, .T. ) ;
#11101=PLANE ( 'NONE',  #1991 ) ;
#11111=CIRCLE ( 'NONE', #1613, 5.425037101889737201 ) ;
#11126=( NAMED_UNIT ( * ) SI_UNIT ( $, .STERADIAN. ) SOLID_ANGLE_UNIT ( ) );
#11152=DIRECTION ( 'NONE',  ( 0.000000000000000000, 0.000000000000000000, -1.000000000000000000 ) ) ;
#11163=ORIENTED_EDGE ( 'NONE', *, *, #11087, .F. ) ;
#11182=CIRCLE ( 'NONE', #19638, 5.425037101889737201 ) ;
#11247=VERTEX_POINT ( 'NONE', #19291 ) ;
#11258=DIRECTION ( 'NONE',  ( 0.5061580162706794672, 0.8624407588727068807, 0.000000000000000000 ) ) ;
#11268=ORIENTED_EDGE ( 'NONE', *, *, #3229, .T. ) ;
#11281=CARTESIAN_POINT ( 'NONE',  ( 161.4980277546683283, 196.8248625098966897, 21.73429951086134082 ) ) ;
#11285=LINE ( 'NONE', #21332, #17506 ) ;
#11371=CARTESIAN_POINT ( 'NONE',  ( 137.5268905834513191, 193.0332408774651185, -44.99999999999997158 ) ) ;
#11373=ORIENTED_EDGE ( 'NONE', *, *, #4463, .T. ) ;
#11435=EDGE_LOOP ( 'NONE', ( #18821, #11689, #9877, #5324, #10643, #13042 ) ) ;
#11533=VECTOR ( 'NONE', #17115, 1000.000000000000000 ) ;
#11534=CARTESIAN_POINT ( 'NONE',  ( 163.3401611601853460, 191.7221236944927796, 21.49552782297503128 ) ) ;
#11666=DIRECTION ( 'NONE',  ( -0.5061580162706792452, -0.8624407588727071028, 0.000000000000000000 ) ) ;
#11668=APPLICATION_CONTEXT ( 'automotive_design' ) ;
#11689=ORIENTED_EDGE ( 'NONE', *, *, #10773, .T. ) ;
#11750=CARTESIAN_POINT ( 'NONE',  ( 163.1026836591718734, 192.4288937294299160, 14.00000000000001776 ) ) ;
#11815=DIRECTION ( 'NONE',  ( -0.7071067811865456854, 8.659560562354910671E-17, 0.7071067811865493491 ) ) ;
#11866=SHAPE_REPRESENTATION_RELATIONSHIP ( 'NONE' , 'NONE' ,  #1720, #20586 ) ;
#11871=AXIS2_PLACEMENT_3D ( 'NONE', #17728, #6053, #5943 ) ;
#11898=VECTOR ( 'NONE', #10339, 1000.000000000000000 ) ;
#11936=EDGE_CURVE ( 'NONE', #6852, #175, #11285, .T. ) ;
#12033=AXIS2_PLACEMENT_3D ( 'NONE', #385, #16606, #8660 ) ;
#12040=ORIENTED_EDGE ( 'NONE', *, *, #3285, .T. ) ;
#12052=CYLINDRICAL_SURFACE ( 'NONE', #12163, 5.425037101889737201 ) ;
#12097=EDGE_CURVE ( 'NONE', #6852, #16883, #378, .T. ) ;
#12146=AXIS2_PLACEMENT_3D ( 'NONE', #20587, #17586, #17371 ) ;
#12163=AXIS2_PLACEMENT_3D ( 'NONE', #20442, #18782, #7002 ) ;
#12175=VECTOR ( 'NONE', #7769, 1000.000000000000000 ) ;
#12191=CARTESIAN_POINT ( 'NONE',  ( 156.7804311855217065, 208.8003142469820830, -44.99999999999997158 ) ) ;
#12199=ORIENTED_EDGE ( 'NONE', *, *, #14114, .T. ) ;
#12257=ORIENTED_EDGE ( 'NONE', *, *, #5437, .T. ) ;
#12264=CARTESIAN_POINT ( 'NONE',  ( 136.1800780017398722, 182.0764489627892715, 20.08191530401613178 ) ) ;
#12283=CIRCLE ( 'NONE', #3856, 10.00000000000000888 ) ;
#12336=VERTEX_POINT ( 'NONE', #17333 ) ;
#12379=VERTEX_POINT ( 'NONE', #21093 ) ;
#12388=CARTESIAN_POINT ( 'NONE',  ( 136.0032066456581390, 182.5367998656340944, 14.00000000000001776 ) ) ;
#12398=CIRCLE ( 'NONE', #20858, 14.42424326798555434 ) ;
#12402=CARTESIAN_POINT ( 'NONE',  ( 136.2275274985377678, 181.9605282764600815, 22.92609503421871864 ) ) ;
#12484=CARTESIAN_POINT ( 'NONE',  ( 136.0836978799983967, 182.3207987053756938, 19.41518736053559024 ) ) ;
#12509=CARTESIAN_POINT ( 'NONE',  ( 163.1026836591718734, 192.4288937294299160, 14.00000000000001776 ) ) ;
#12513=CARTESIAN_POINT ( 'NONE',  ( 136.0032066456581390, 182.5367998656340944, 24.47866928663567521 ) ) ;
#12554=ORIENTED_EDGE ( 'NONE', *, *, #3935, .T. ) ;
#12566=PLANE ( 'NONE',  #8442 ) ;
#12589=AXIS2_PLACEMENT_3D ( 'NONE', #14144, #10308, #8440 ) ;
#12636=CARTESIAN_POINT ( 'NONE',  ( 0.000000000000000000, 0.000000000000000000, -29.99999999999997868 ) ) ;
#12657=AXIS2_PLACEMENT_3D ( 'NONE', #2403, #7050, #17169 ) ;
#12688=ORIENTED_EDGE ( 'NONE', *, *, #10518, .T. ) ;
#12712=DIRECTION ( 'NONE',  ( 0.000000000000000000, 0.000000000000000000, -1.000000000000000000 ) ) ;
#12728=DIRECTION ( 'NONE',  ( 0.3428981916074316239, -0.9393725726208708160, -0.000000000000000000 ) ) ;
#12794=VERTEX_POINT ( 'NONE', #8367 ) ;
#12851=VERTEX_POINT ( 'NONE', #3407 ) ;
#12893=DIRECTION ( 'NONE',  ( 1.000000000000000000, 0.000000000000000000, -0.000000000000000000 ) ) ;
#12894=CARTESIAN_POINT ( 'NONE',  ( 165.8083469658213005, 192.9029763258799335, -44.99999999999997158 ) ) ;
#12914=CARTESIAN_POINT ( 'NONE',  ( 156.7804311855217065, 208.8003142469820830, -44.99999999999997158 ) ) ;
#12968=DIRECTION ( 'NONE',  ( -0.000000000000000000, -0.000000000000000000, -1.000000000000000000 ) ) ;
#12990=VECTOR ( 'NONE', #7906, 1000.000000000000114 ) ;
#13042=ORIENTED_EDGE ( 'NONE', *, *, #2304, .T. ) ;
#13076=FACE_OUTER_BOUND ( 'NONE', #15614, .T. ) ;
#13108=CARTESIAN_POINT ( 'NONE',  ( 137.5268905834513191, 193.0332408774651185, -50.99999999999998579 ) ) ;
#13158=ORIENTED_EDGE ( 'NONE', *, *, #6789, .T. ) ;
#13253=CARTESIAN_POINT ( 'NONE',  ( 129.2454342010813662, 193.1635054290503319, -44.99999999999997158 ) ) ;
#13315=DIRECTION ( 'NONE',  ( 1.000000000000000000, 0.000000000000000000, 0.000000000000000000 ) ) ;
#13363=CARTESIAN_POINT ( 'NONE',  ( 157.5268905834513475, 193.0332408774651185, -49.99999999999997158 ) ) ;
#13364=DIRECTION ( 'NONE',  ( 0.4938165983075534227, -0.8695660798558993987, 0.000000000000000000 ) ) ;
#13383=CLOSED_SHELL ( 'NONE', ( #13551, #16106, #5631, #20806, #19190, #8936, #9175, #7500, #2284, #14826, #1115, #18913, #2105, #6871, #1061, #4837, #5099, #9999, #7228, #6963, #7645, #18414, #5033, #1739 ) ) ;
#13551=ADVANCED_FACE ( 'NONE', ( #3895 ), #14999, .T. ) ;
#13585=VERTEX_POINT ( 'NONE', #4000 ) ;
#13606=CARTESIAN_POINT ( 'NONE',  ( 163.1026836591718734, 192.4288937294299160, 34.00000000000001421 ) ) ;
#13651=FACE_OUTER_BOUND ( 'NONE', #14873, .T. ) ;
#13681=DIRECTION ( 'NONE',  ( 1.000000000000000000, 0.000000000000000000, 0.000000000000000000 ) ) ;
#13707=CARTESIAN_POINT ( 'NONE',  ( 136.2768881589198884, 181.8432453435730167, 21.73429951086134082 ) ) ;
#13769=ORIENTED_EDGE ( 'NONE', *, *, #18244, .F. ) ;
#13771=LINE ( 'NONE', #5610, #5012 ) ;
#13785=CARTESIAN_POINT ( 'NONE',  ( 175.9120630731088397, 202.0864028065961122, 21.73429951086134082 ) ) ;
#13800=AXIS2_PLACEMENT_3D ( 'NONE', #13785, #20524, #15768 ) ;
#13920=EDGE_CURVE ( 'NONE', #14777, #9423, #1122, .T. ) ;
#13940=CARTESIAN_POINT ( 'NONE',  ( 163.1802725128760585, 192.2118331161914568, 24.05341166118710561 ) ) ;
#13944=DIRECTION ( 'NONE',  ( 1.000000000000000000, 0.000000000000000000, 0.000000000000000000 ) ) ;
#14047=AXIS2_PLACEMENT_3D ( 'NONE', #21716, #1429, #9922 ) ;
#14108=CARTESIAN_POINT ( 'NONE',  ( 159.0505745212445561, 203.5296818892961994, 34.00000000000001421 ) ) ;
#14111=ORIENTED_EDGE ( 'NONE', *, *, #3646, .T. ) ;
#14114=EDGE_CURVE ( 'NONE', #175, #12379, #15050, .T. ) ;
#14124=DIRECTION ( 'NONE',  ( 0.000000000000000000, 0.000000000000000000, 1.000000000000000000 ) ) ;
#14144=CARTESIAN_POINT ( 'NONE',  ( 129.2454342010813662, 193.1635054290503319, -44.99999999999997158 ) ) ;
#14232=CARTESIAN_POINT ( 'NONE',  ( 147.5268905834513475, 193.0332408774651185, -50.99999999999998579 ) ) ;
#14246=VERTEX_POINT ( 'NONE', #7554 ) ;
#14274=ORIENTED_EDGE ( 'NONE', *, *, #5860, .F. ) ;
#14301=CARTESIAN_POINT ( 'NONE',  ( 138.2733499813809885, 177.2661675079481540, -44.99999999999997158 ) ) ;
#14309=VERTEX_POINT ( 'NONE', #16013 ) ;
#14318=EDGE_CURVE ( 'NONE', #4323, #1933, #2573, .T. ) ;
#14364=ORIENTED_EDGE ( 'NONE', *, *, #17674, .T. ) ;
#14397=CARTESIAN_POINT ( 'NONE',  ( 145.5008360144876747, 198.5836349573982886, 34.00000000000001421 ) ) ;
#14414=CARTESIAN_POINT ( 'NONE',  ( 149.5529451524149920, 187.4828467975320336, 34.00000000000001421 ) ) ;
#14485=AXIS2_PLACEMENT_3D ( 'NONE', #410, #5151, #17149 ) ;
#14522=CARTESIAN_POINT ( 'NONE',  ( 147.5268905834513475, 193.0332408774651185, -49.99999999999997158 ) ) ;
#14634=ORIENTED_EDGE ( 'NONE', *, *, #9508, .F. ) ;
#14645=VECTOR ( 'NONE', #8812, 1000.000000000000114 ) ;
#14650=CARTESIAN_POINT ( 'NONE',  ( 134.3985507411545939, 186.9327686461008682, 21.73429951086134082 ) ) ;
#14722=EDGE_CURVE ( 'NONE', #12379, #1227, #13771, .T. ) ;
#14774=ORIENTED_EDGE ( 'NONE', *, *, #1256, .F. ) ;
#14777=VERTEX_POINT ( 'NONE', #17401 ) ;
#14796=CARTESIAN_POINT ( 'NONE',  ( 165.8083469658213005, 192.9029763258799335, -44.99999999999997158 ) ) ;
#14826=ADVANCED_FACE ( 'NONE', ( #15754 ), #2303, .F. ) ;
#14862=DIRECTION ( 'NONE',  ( -0.8624407588727071028, 0.5061580162706792452, 0.000000000000000000 ) ) ;
#14873=EDGE_LOOP ( 'NONE', ( #9996, #2461, #14111, #6723 ) ) ;
#14896=ORIENTED_EDGE ( 'NONE', *, *, #18208, .T. ) ;
#14993=PRODUCT ( 'Blade Pivot Hinge Pin', 'Blade Pivot Hinge Pin', '', ( #6000 ) ) ;
#14999=CONICAL_SURFACE ( 'NONE', #3404, 9.000000000000007105, 0.7853981633974457255 ) ;
#15032=PLANE ( 'NONE',  #91 ) ;
#15050=LINE ( 'NONE', #15162, #6202 ) ;
#15099=DIRECTION ( 'NONE',  ( -0.4938165983075539223, 0.8695660798558991766, 0.000000000000000000 ) ) ;
#15105=EDGE_LOOP ( 'NONE', ( #3906, #17475 ) ) ;
#15135=VERTEX_POINT ( 'NONE', #5020 ) ;
#15143=PRESENTATION_STYLE_ASSIGNMENT (( #3248 ) ) ;
#15162=CARTESIAN_POINT ( 'NONE',  ( 129.2454342010813662, 193.1635054290503319, -44.99999999999997158 ) ) ;
#15174=DIRECTION ( 'NONE',  ( -0.9393725726208707050, -0.3428981916074316239, -0.000000000000000000 ) ) ;
#15188=DIRECTION ( 'NONE',  ( -1.000000000000000000, 0.000000000000000000, 0.000000000000000000 ) ) ;
#15222=AXIS2_PLACEMENT_3D ( 'NONE', #14522, #6368, #9474 ) ;
#15224=EDGE_LOOP ( 'NONE', ( #2569, #16701, #6671, #13158 ) ) ;
#15227=AXIS2_PLACEMENT_3D ( 'NONE', #1812, #15370, #6787 ) ;
#15327=VECTOR ( 'NONE', #17034, 1000.000000000000114 ) ;
#15351=EDGE_CURVE ( 'NONE', #5871, #15900, #4008, .T. ) ;
#15354=APPLICATION_CONTEXT ( 'automotive_design' ) ;
#15370=DIRECTION ( 'NONE',  ( 0.007125320983193088667, 0.9999746145782334450, 0.000000000000000000 ) ) ;
#15396=LINE ( 'NONE', #3384, #1123 ) ;
#15413=ORIENTED_EDGE ( 'NONE', *, *, #8231, .F. ) ;
#15502=LINE ( 'NONE', #180, #1948 ) ;
#15526=DIRECTION ( 'NONE',  ( 1.000000000000000000, 0.000000000000000000, 0.000000000000000000 ) ) ;
#15578=PLANE ( 'NONE',  #2715 ) ;
#15614=EDGE_LOOP ( 'NONE', ( #1418, #8977, #3237, #5792 ) ) ;
#15625=DIRECTION ( 'NONE',  ( -0.000000000000000000, -0.000000000000000000, 1.000000000000000000 ) ) ;
#15633=DIRECTION ( 'NONE',  ( 1.000000000000000000, 0.000000000000000000, 0.000000000000000000 ) ) ;
#15655=CYLINDRICAL_SURFACE ( 'NONE', #13800, 5.425037101889737201 ) ;
#15687=DIRECTION ( 'NONE',  ( -0.000000000000000000, -0.000000000000000000, -1.000000000000000000 ) ) ;
#15689=VECTOR ( 'NONE', #2806, 1000.000000000000000 ) ;
#15692=EDGE_CURVE ( 'NONE', #14309, #8397, #18864, .T. ) ;
#15754=FACE_OUTER_BOUND ( 'NONE', #17023, .T. ) ;
#15768=DIRECTION ( 'NONE',  ( 0.3428981916074309577, -0.9393725726208709270, 0.000000000000000000 ) ) ;
#15778=ORIENTED_EDGE ( 'NONE', *, *, #1462, .T. ) ;
#15786=CARTESIAN_POINT ( 'NONE',  ( 136.2768881589198884, 181.8432453435730451, 21.25738000485995016 ) ) ;
#15788=CARTESIAN_POINT ( 'NONE',  ( 147.5268905834513475, 193.0332408774651185, -50.99999999999998579 ) ) ;
#15825=PLANE ( 'NONE',  #12146 ) ;
#15830=EDGE_CURVE ( 'NONE', #14246, #15135, #8524, .T. ) ;
#15892=VECTOR ( 'NONE', #7224, 1000.000000000000000 ) ;
#15900=VERTEX_POINT ( 'NONE', #10281 ) ;
#15952=PLANE ( 'NONE',  #6130 ) ;
#15996=CARTESIAN_POINT ( 'NONE',  ( 147.5268905834513475, 193.0332408774651185, -50.99999999999998579 ) ) ;
#16013=CARTESIAN_POINT ( 'NONE',  ( 138.5268905834513191, 193.0332408774651185, -50.99999999999998579 ) ) ;
#16106=ADVANCED_FACE ( 'NONE', ( #18269 ), #20559, .T. ) ;
#16114=FACE_OUTER_BOUND ( 'NONE', #5740, .T. ) ;
#16132=EDGE_CURVE ( 'NONE', #2768, #6540, #17227, .T. ) ;
#16154=ORIENTED_EDGE ( 'NONE', *, *, #5437, .F. ) ;
#16261=AXIS2_PLACEMENT_3D ( 'NONE', #765, #20831, #2096 ) ;
#16274=CARTESIAN_POINT ( 'NONE',  ( 163.3401611601854029, 191.7221236944928364, 21.73429951086134082 ) ) ;
#16333=EDGE_CURVE ( 'NONE', #497, #4860, #3587, .T. ) ;
#16339=AXIS2_PLACEMENT_3D ( 'NONE', #1813, #9080, #692 ) ;
#16415=VERTEX_POINT ( 'NONE', #5242 ) ;
#16425=ORIENTED_EDGE ( 'NONE', *, *, #10773, .F. ) ;
#16432=DIRECTION ( 'NONE',  ( -1.000000000000000000, 0.000000000000000000, -0.000000000000000000 ) ) ;
#16448=EDGE_LOOP ( 'NONE', ( #2124, #11163, #2667, #16811 ) ) ;
#16456=FACE_OUTER_BOUND ( 'NONE', #19070, .T. ) ;
#16553=ORIENTED_EDGE ( 'NONE', *, *, #5276, .F. ) ;
#16558=ORIENTED_EDGE ( 'NONE', *, *, #3467, .F. ) ;
#16602=B_SPLINE_CURVE_WITH_KNOTS ( 'NONE', 3,
 ( #9568, #9894, #21466, #4699, #6707, #18142, #11534, #16274 ),
 .UNSPECIFIED., .F., .F.,
 ( 4, 2, 2, 4 ),
 ( 3.469446951953614189E-18, 0.001432241572422958973, 0.002148362358634439868, 0.002864483144845920981 ),
 .UNSPECIFIED. ) ;
#16606=DIRECTION ( 'NONE',  ( -0.000000000000000000, -0.000000000000000000, 1.000000000000000000 ) ) ;
#16648=VERTEX_POINT ( 'NONE', #12388 ) ;
#16678=EDGE_CURVE ( 'NONE', #15135, #17794, #20881, .T. ) ;
#16701=ORIENTED_EDGE ( 'NONE', *, *, #5344, .F. ) ;
#16724=CONICAL_SURFACE ( 'NONE', #10059, 9.000000000000007105, 0.7853981633974457255 ) ;
#16748=CARTESIAN_POINT ( 'NONE',  ( 138.2733499813809885, 177.2661675079481540, -29.99999999999997868 ) ) ;
#16754=EDGE_LOOP ( 'NONE', ( #4304, #8507, #14274, #8068, #9173 ) ) ;
#16792=DIRECTION ( 'NONE',  ( 0.000000000000000000, 0.000000000000000000, -1.000000000000000000 ) ) ;
#16793=LINE ( 'NONE', #18567, #1211 ) ;
#16802=VECTOR ( 'NONE', #9170, 1000.000000000000000 ) ;
#16811=ORIENTED_EDGE ( 'NONE', *, *, #980, .T. ) ;
#16864=CIRCLE ( 'NONE', #14047, 9.000000000000007105 ) ;
#16883=VERTEX_POINT ( 'NONE', #2463 ) ;
#16899=FACE_OUTER_BOUND ( 'NONE', #4658, .T. ) ;
#16952=VECTOR ( 'NONE', #7770, 1000.000000000000227 ) ;
#17017=CARTESIAN_POINT ( 'NONE',  ( 131.0765927465021434, 198.5836349573982886, 34.00000000000001421 ) ) ;
#17023=EDGE_LOOP ( 'NONE', ( #149, #10344, #20459, #3861, #2488, #6261, #8400 ) ) ;
#17034=DIRECTION ( 'NONE',  ( -0.3428981916074316239, 0.9393725726208708160, 0.000000000000000000 ) ) ;
#17115=DIRECTION ( 'NONE',  ( -0.000000000000000000, -0.000000000000000000, 1.000000000000000000 ) ) ;
#17149=DIRECTION ( 'NONE',  ( 1.000000000000000000, 0.000000000000000000, 0.000000000000000000 ) ) ;
#17169=DIRECTION ( 'NONE',  ( 1.000000000000000000, 0.000000000000000000, 0.000000000000000000 ) ) ;
#17193=B_SPLINE_CURVE_WITH_KNOTS ( 'NONE', 3,
 ( #8972, #15786, #20653, #12264, #5755, #12484, #5651, #10521 ),
 .UNSPECIFIED., .F., .F.,
 ( 4, 2, 2, 4 ),
 ( 0.002864483144845920114, 0.004294853615569176747, 0.005010038850930815038, 0.005725224086292454197 ),
 .UNSPECIFIED. ) ;
#17227=LINE ( 'NONE', #13606, #15892 ) ;
#17304=DIRECTION ( 'NONE',  ( -1.000000000000000000, 0.000000000000000000, 0.000000000000000000 ) ) ;
#17333=CARTESIAN_POINT ( 'NONE',  ( 156.5548063637509415, 177.1359029563629406, -44.99999999999997158 ) ) ;
#17334=DIRECTION ( 'NONE',  ( 1.000000000000000000, 0.000000000000000000, 0.000000000000000000 ) ) ;
#17354=CARTESIAN_POINT ( 'NONE',  ( 163.2398440670430944, 192.0365442723309570, 23.61216616543570979 ) ) ;
#17371=DIRECTION ( 'NONE',  ( 1.000000000000000000, 0.000000000000000000, -0.000000000000000000 ) ) ;
#17393=DIRECTION ( 'NONE',  ( 0.000000000000000000, 0.000000000000000000, 1.000000000000000000 ) ) ;
#17401=CARTESIAN_POINT ( 'NONE',  ( 156.7804311855217065, 208.8003142469820830, -44.99999999999997158 ) ) ;
#17414=DIRECTION ( 'NONE',  ( 0.000000000000000000, 0.000000000000000000, -1.000000000000000000 ) ) ;
#17428=EDGE_CURVE ( 'NONE', #16883, #10216, #18416, .T. ) ;
#17464=CARTESIAN_POINT ( 'NONE',  ( 136.2707191487307341, 181.8577005505615034, 22.21145758847113427 ) ) ;
#17475=ORIENTED_EDGE ( 'NONE', *, *, #3646, .F. ) ;
#17506=VECTOR ( 'NONE', #3026, 1000.000000000000000 ) ;
#17526=ORIENTED_EDGE ( 'NONE', *, *, #1386, .F. ) ;
#17572=DIRECTION ( 'NONE',  ( 0.000000000000000000, 0.000000000000000000, 1.000000000000000000 ) ) ;
#17586=DIRECTION ( 'NONE',  ( 0.000000000000000000, 0.000000000000000000, 1.000000000000000000 ) ) ;
#17606=DIRECTION ( 'NONE',  ( -0.4938165983075539223, 0.8695660798558990656, 0.000000000000000000 ) ) ;
#17674=EDGE_CURVE ( 'NONE', #12379, #14777, #439, .T. ) ;
#17675=B_SPLINE_CURVE_WITH_KNOTS ( 'NONE', 3,
 ( #4835, #5563, #3921, #7452, #17354, #13940, #19131, #10755 ),
 .UNSPECIFIED., .F., .F.,
 ( 4, 2, 2, 4 ),
 ( 0.002864483144845920981, 0.004294853615569181084, 0.005010038850930821110, 0.005725224086292461136 ),
 .UNSPECIFIED. ) ;
#17728=CARTESIAN_POINT ( 'NONE',  ( 147.5268905834513475, 193.0332408774651185, -29.99999999999997868 ) ) ;
#17735=DIRECTION ( 'NONE',  ( -0.000000000000000000, -0.000000000000000000, 1.000000000000000000 ) ) ;
#17761=CARTESIAN_POINT ( 'NONE',  ( 134.3985507411545939, 186.9327686461008682, 21.73429951086134082 ) ) ;
#17785=CARTESIAN_POINT ( 'NONE',  ( 136.2461330483349968, 181.9161108113851526, 22.68744729171066155 ) ) ;
#17794=VERTEX_POINT ( 'NONE', #973 ) ;
#17814=DIRECTION ( 'NONE',  ( 0.4938165983075534782, -0.8695660798558993987, 0.000000000000000000 ) ) ;
#17819=DIRECTION ( 'NONE',  ( 0.8695660798558991766, 0.4938165983075539778, 0.000000000000000000 ) ) ;
#17876=ORIENTED_EDGE ( 'NONE', *, *, #17887, .F. ) ;
#17887=EDGE_CURVE ( 'NONE', #5468, #8397, #7126, .T. ) ;
#17950=PLANE ( 'NONE',  #6484 ) ;
#17999=VECTOR ( 'NONE', #13364, 1000.000000000000114 ) ;
#18001=LINE ( 'NONE', #3133, #9407 ) ;
#18090=FACE_OUTER_BOUND ( 'NONE', #16448, .T. ) ;
#18092=DIRECTION ( 'NONE',  ( 0.3428981916074309577, -0.9393725726208709270, 0.000000000000000000 ) ) ;
#18099=VERTEX_POINT ( 'NONE', #5015 ) ;
#18142=CARTESIAN_POINT ( 'NONE',  ( 163.3355671671241680, 191.7371538283428265, 21.25714143325154026 ) ) ;
#18152=CIRCLE ( 'NONE', #8670, 14.42424326798555434 ) ;
#18190=CIRCLE ( 'NONE', #11871, 10.00000000000000888 ) ;
#18208=EDGE_CURVE ( 'NONE', #10265, #5468, #16793, .T. ) ;
#18228=EDGE_CURVE ( 'NONE', #8397, #5468, #10368, .T. ) ;
#18232=DIRECTION ( 'NONE',  ( 0.000000000000000000, 0.000000000000000000, 1.000000000000000000 ) ) ;
#18244=EDGE_CURVE ( 'NONE', #2204, #1699, #17193, .T. ) ;
#18269=FACE_OUTER_BOUND ( 'NONE', #21517, .T. ) ;
#18307=ORIENTED_EDGE ( 'NONE', *, *, #18244, .T. ) ;
#18323=DIRECTION ( 'NONE',  ( -0.000000000000000000, -0.000000000000000000, 1.000000000000000000 ) ) ;
#18414=ADVANCED_FACE ( 'NONE', ( #16114 ), #2887, .T. ) ;
#18416=LINE ( 'NONE', #16748, #18728 ) ;
#18432=DIRECTION ( 'NONE',  ( -0.000000000000000000, -0.000000000000000000, 1.000000000000000000 ) ) ;
#18456=FILL_AREA_STYLE ('',( #155 ) ) ;
#18533=EDGE_CURVE ( 'NONE', #12336, #17794, #5095, .T. ) ;
#18567=CARTESIAN_POINT ( 'NONE',  ( 156.5268905834513475, 193.0332408774651185, -50.99999999999998579 ) ) ;
#18569=CARTESIAN_POINT ( 'NONE',  ( 138.2733499813809885, 177.2661675079481540, -44.99999999999997158 ) ) ;
#18728=VECTOR ( 'NONE', #15099, 1000.000000000000000 ) ;
#18760=DIRECTION ( 'NONE',  ( -0.000000000000000000, -0.000000000000000000, -1.000000000000000000 ) ) ;
#18782=DIRECTION ( 'NONE',  ( -0.9393725726208707050, -0.3428981916074316794, -0.000000000000000000 ) ) ;
#18796=ORIENTED_EDGE ( 'NONE', *, *, #18228, .T. ) ;
#18821=ORIENTED_EDGE ( 'NONE', *, *, #14318, .F. ) ;
#18864=LINE ( 'NONE', #3661, #7125 ) ;
#18905=ORIENTED_EDGE ( 'NONE', *, *, #10518, .F. ) ;
#18913=ADVANCED_FACE ( 'NONE', ( #9167, #883 ), #17950, .F. ) ;
#18955=DIRECTION ( 'NONE',  ( 0.9999746145782334450, -0.007125320983191549967, 0.000000000000000000 ) ) ;
#18962=ORIENTED_EDGE ( 'NONE', *, *, #14722, .T. ) ;
#18990=ORIENTED_EDGE ( 'NONE', *, *, #3935, .F. ) ;
#19070=EDGE_LOOP ( 'NONE', ( #12199, #14364, #19230, #15778, #11268, #9016 ) ) ;
#19072=VECTOR ( 'NONE', #7329, 1000.000000000000000 ) ;
#19084=CYLINDRICAL_SURFACE ( 'NONE', #3810, 14.42424326798555434 ) ;
#19086=CARTESIAN_POINT ( 'NONE',  ( 157.5268905834513475, 193.0332408774651185, -50.99999999999998579 ) ) ;
#19131=CARTESIAN_POINT ( 'NONE',  ( 163.1446318037170897, 192.3139764232951734, 24.27006575478477757 ) ) ;
#19134=CARTESIAN_POINT ( 'NONE',  ( 136.2768881589198884, 181.8432453435730167, 21.73429951086134082 ) ) ;
#19190=ADVANCED_FACE ( 'NONE', ( #13651 ), #430, .T. ) ;
#19230=ORIENTED_EDGE ( 'NONE', *, *, #13920, .T. ) ;
#19251=CIRCLE ( 'NONE', #4817, 5.425037101889737201 ) ;
#19291=CARTESIAN_POINT ( 'NONE',  ( 157.5268905834513475, 193.0332408774651185, -29.99999999999997868 ) ) ;
#19298=LINE ( 'NONE', #19086, #16802 ) ;
#19320=DIRECTION ( 'NONE',  ( -0.000000000000000000, -0.000000000000000000, 1.000000000000000000 ) ) ;
#19322=ORIENTED_EDGE ( 'NONE', *, *, #7348, .F. ) ;
#19357=DIRECTION ( 'NONE',  ( 0.000000000000000000, 0.000000000000000000, -1.000000000000000000 ) ) ;
#19447=DIRECTION ( 'NONE',  ( 1.000000000000000000, 0.000000000000000000, 0.000000000000000000 ) ) ;
#19452=CARTESIAN_POINT ( 'NONE',  ( 136.0872141950132175, 182.3066604549029819, 24.06090893781343709 ) ) ;
#19511=AXIS2_PLACEMENT_3D ( 'NONE', #1864, #3420, #10142 ) ;
#19517=ORIENTED_EDGE ( 'NONE', *, *, #4463, .F. ) ;
#19574=AXIS2_PLACEMENT_3D ( 'NONE', #2674, #12712, #4329 ) ;
#19594=VECTOR ( 'NONE', #9102, 1000.000000000000341 ) ;
#19638=AXIS2_PLACEMENT_3D ( 'NONE', #6690, #8333, #9989 ) ;
#19682=DIRECTION ( 'NONE',  ( 0.000000000000000000, 0.000000000000000000, -1.000000000000000000 ) ) ;
#19825=VERTEX_POINT ( 'NONE', #11371 ) ;
#19844=ORIENTED_EDGE ( 'NONE', *, *, #16678, .F. ) ;
#19853=ORIENTED_EDGE ( 'NONE', *, *, #6437, .F. ) ;
#19869=DIRECTION ( 'NONE',  ( 1.000000000000000000, 0.000000000000000000, 0.000000000000000000 ) ) ;
#19887=EDGE_LOOP ( 'NONE', ( #4094, #21374, #1774, #13769, #17526, #14774 ) ) ;
#19907=CIRCLE ( 'NONE', #6901, 10.00000000000000888 ) ;
#19956=AXIS2_PLACEMENT_3D ( 'NONE', #14414, #17393, #15633 ) ;
#19983=CIRCLE ( 'NONE', #3785, 9.000000000000007105 ) ;
#20018=LINE ( 'NONE', #21442, #15689 ) ;
#20034=ORIENTED_EDGE ( 'NONE', *, *, #18208, .F. ) ;
#20125=CARTESIAN_POINT ( 'NONE',  ( 131.0765927465021434, 198.5836349573982886, 14.00000000000001776 ) ) ;
#20217=ORIENTED_EDGE ( 'NONE', *, *, #7944, .T. ) ;
#20292=VERTEX_POINT ( 'NONE', #1420 ) ;
#20323=EDGE_CURVE ( 'NONE', #20292, #11247, #12283, .T. ) ;
#20336=UNCERTAINTY_MEASURE_WITH_UNIT (LENGTH_MEASURE( 1.000000000000000082E-05 ), #21579, 'distance_accuracy_value', 'NONE');
#20357=DIRECTION ( 'NONE',  ( -0.000000000000000000, -0.000000000000000000, -1.000000000000000000 ) ) ;
#20361=( GEOMETRIC_REPRESENTATION_CONTEXT ( 3 ) GLOBAL_UNCERTAINTY_ASSIGNED_CONTEXT ( ( #7539 ) ) GLOBAL_UNIT_ASSIGNED_CONTEXT ( ( #5118, #9270, #11126 ) ) REPRESENTATION_CONTEXT ( 'NONE', 'WORKASPACE' ) );
#20385=CARTESIAN_POINT ( 'NONE',  ( 147.5268905834513475, 193.0332408774651185, -50.99999999999998579 ) ) ;
#20415=CARTESIAN_POINT ( 'NONE',  ( 136.0032066456581390, 182.5367998656340944, 34.00000000000001421 ) ) ;
#20418=VERTEX_POINT ( 'NONE', #6608 ) ;
#20442=CARTESIAN_POINT ( 'NONE',  ( 175.9120630731088397, 202.0864028065961122, 21.73429951086134082 ) ) ;
#20458=DIRECTION ( 'NONE',  ( 0.5061580162706794672, 0.8624407588727068807, 0.000000000000000000 ) ) ;
#20459=ORIENTED_EDGE ( 'NONE', *, *, #2304, .F. ) ;
#20524=DIRECTION ( 'NONE',  ( -0.9393725726208707050, -0.3428981916074316794, -0.000000000000000000 ) ) ;
#20528=ORIENTED_EDGE ( 'NONE', *, *, #17428, .F. ) ;
#20559=CYLINDRICAL_SURFACE ( 'NONE', #12033, 10.00000000000000888 ) ;
#20586=ADVANCED_BREP_SHAPE_REPRESENTATION ( '', ( #7102, #12657 ), #4220 ) ;
#20587=CARTESIAN_POINT ( 'NONE',  ( 149.5529451524149920, 187.4828467975320336, 34.00000000000001421 ) ) ;
#20618=ORIENTED_EDGE ( 'NONE', *, *, #3330, .T. ) ;
#20627=AXIS2_PLACEMENT_3D ( 'NONE', #20955, #9381, #886 ) ;
#20653=CARTESIAN_POINT ( 'NONE',  ( 136.2512292229016566, 181.9026294830433699, 20.77285216529425682 ) ) ;
#20655=EDGE_CURVE ( 'NONE', #5468, #12794, #2499, .T. ) ;
#20695=PLANE ( 'NONE',  #7585 ) ;
#20697=ORIENTED_EDGE ( 'NONE', *, *, #13920, .F. ) ;
#20750=AXIS2_PLACEMENT_3D ( 'NONE', #14397, #12968, #4261 ) ;
#20764=VECTOR ( 'NONE', #4721, 1000.000000000000000 ) ;
#20787=FACE_OUTER_BOUND ( 'NONE', #21155, .T. ) ;
#20806=ADVANCED_FACE ( 'NONE', ( #13076 ), #1395, .T. ) ;
#20831=DIRECTION ( 'NONE',  ( 0.9393725726208708160, 0.3428981916074316239, -0.000000000000000000 ) ) ;
#20858=AXIS2_PLACEMENT_3D ( 'NONE', #9759, #18232, #19447 ) ;
#20870=EDGE_CURVE ( 'NONE', #1227, #14246, #4582, .T. ) ;
#20873=ORIENTED_EDGE ( 'NONE', *, *, #1561, .T. ) ;
#20881=LINE ( 'NONE', #4330, #16952 ) ;
#20884=ORIENTED_EDGE ( 'NONE', *, *, #17887, .T. ) ;
#20914=ORIENTED_EDGE ( 'NONE', *, *, #16678, .T. ) ;
#20916=DIRECTION ( 'NONE',  ( -0.000000000000000000, -0.000000000000000000, 1.000000000000000000 ) ) ;
#20928=FACE_OUTER_BOUND ( 'NONE', #5221, .T. ) ;
#20955=CARTESIAN_POINT ( 'NONE',  ( 145.5008360144876747, 198.5836349573982886, 34.00000000000001421 ) ) ;
#20980=FACE_OUTER_BOUND ( 'NONE', #4829, .T. ) ;
#20983=CIRCLE ( 'NONE', #5417, 14.42424326798555434 ) ;
#21065=CARTESIAN_POINT ( 'NONE',  ( 149.5529451524149920, 187.4828467975320336, 14.00000000000001776 ) ) ;
#21093=CARTESIAN_POINT ( 'NONE',  ( 138.4989748031516967, 208.9305787985672680, -44.99999999999997158 ) ) ;
#21155=EDGE_LOOP ( 'NONE', ( #445, #19517, #14896, #3540 ) ) ;
#21159=DIRECTION ( 'NONE',  ( 0.000000000000000000, 0.000000000000000000, -1.000000000000000000 ) ) ;
#21182=ORIENTED_EDGE ( 'NONE', *, *, #18533, .T. ) ;
#21197=LINE ( 'NONE', #6083, #612 ) ;
#21259=FACE_OUTER_BOUND ( 'NONE', #369, .T. ) ;
#21332=CARTESIAN_POINT ( 'NONE',  ( 138.2733499813809885, 177.2661675079481540, -44.99999999999997158 ) ) ;
#21374=ORIENTED_EDGE ( 'NONE', *, *, #14318, .T. ) ;
#21390=DIRECTION ( 'NONE',  ( 0.3428981916074309577, -0.9393725726208709270, 0.000000000000000000 ) ) ;
#21413=STYLED_ITEM ( 'NONE', ( #15143 ), #7102 ) ;
#21427=LINE ( 'NONE', #14796, #12175 ) ;
#21442=CARTESIAN_POINT ( 'NONE',  ( 131.9510975077307933, 193.6375880255003779, 34.00000000000001421 ) ) ;
#21452=DIRECTION ( 'NONE',  ( -1.000000000000000000, 0.000000000000000000, 0.000000000000000000 ) ) ;
#21466=CARTESIAN_POINT ( 'NONE',  ( 163.2444732741424787, 192.0234091111227883, 19.84828153075611823 ) ) ;
#21477=EDGE_CURVE ( 'NONE', #20292, #12851, #6379, .T. ) ;
#21484=EDGE_CURVE ( 'NONE', #6341, #18099, #17675, .T. ) ;
#21517=EDGE_LOOP ( 'NONE', ( #20884, #6752, #93, #7767 ) ) ;
#21532=ORIENTED_EDGE ( 'NONE', *, *, #17428, .T. ) ;
#21579=( LENGTH_UNIT ( ) NAMED_UNIT ( * ) SI_UNIT ( .MILLI., .METRE. ) );
#21639=CARTESIAN_POINT ( 'NONE',  ( 147.5268905834513475, 193.0332408774651185, -50.99999999999998579 ) ) ;
#21674=CARTESIAN_POINT ( 'NONE',  ( 137.5268905834513191, 193.0332408774651185, -49.99999999999997158 ) ) ;
#21697=DIRECTION ( 'NONE',  ( 1.000000000000000000, 0.000000000000000000, 0.000000000000000000 ) ) ;
#21716=CARTESIAN_POINT ( 'NONE',  ( 147.5268905834513475, 193.0332408774651185, -50.99999999999998579 ) ) ;
#21741=AXIS2_PLACEMENT_3D ( 'NONE', #6763, #237, #13681 ) ;
#21775=FACE_OUTER_BOUND ( 'NONE', #11435, .T. ) ;
#21795=LINE ( 'NONE', #291, #583 ) ;
ENDSEC;
END-ISO-10303-21;
